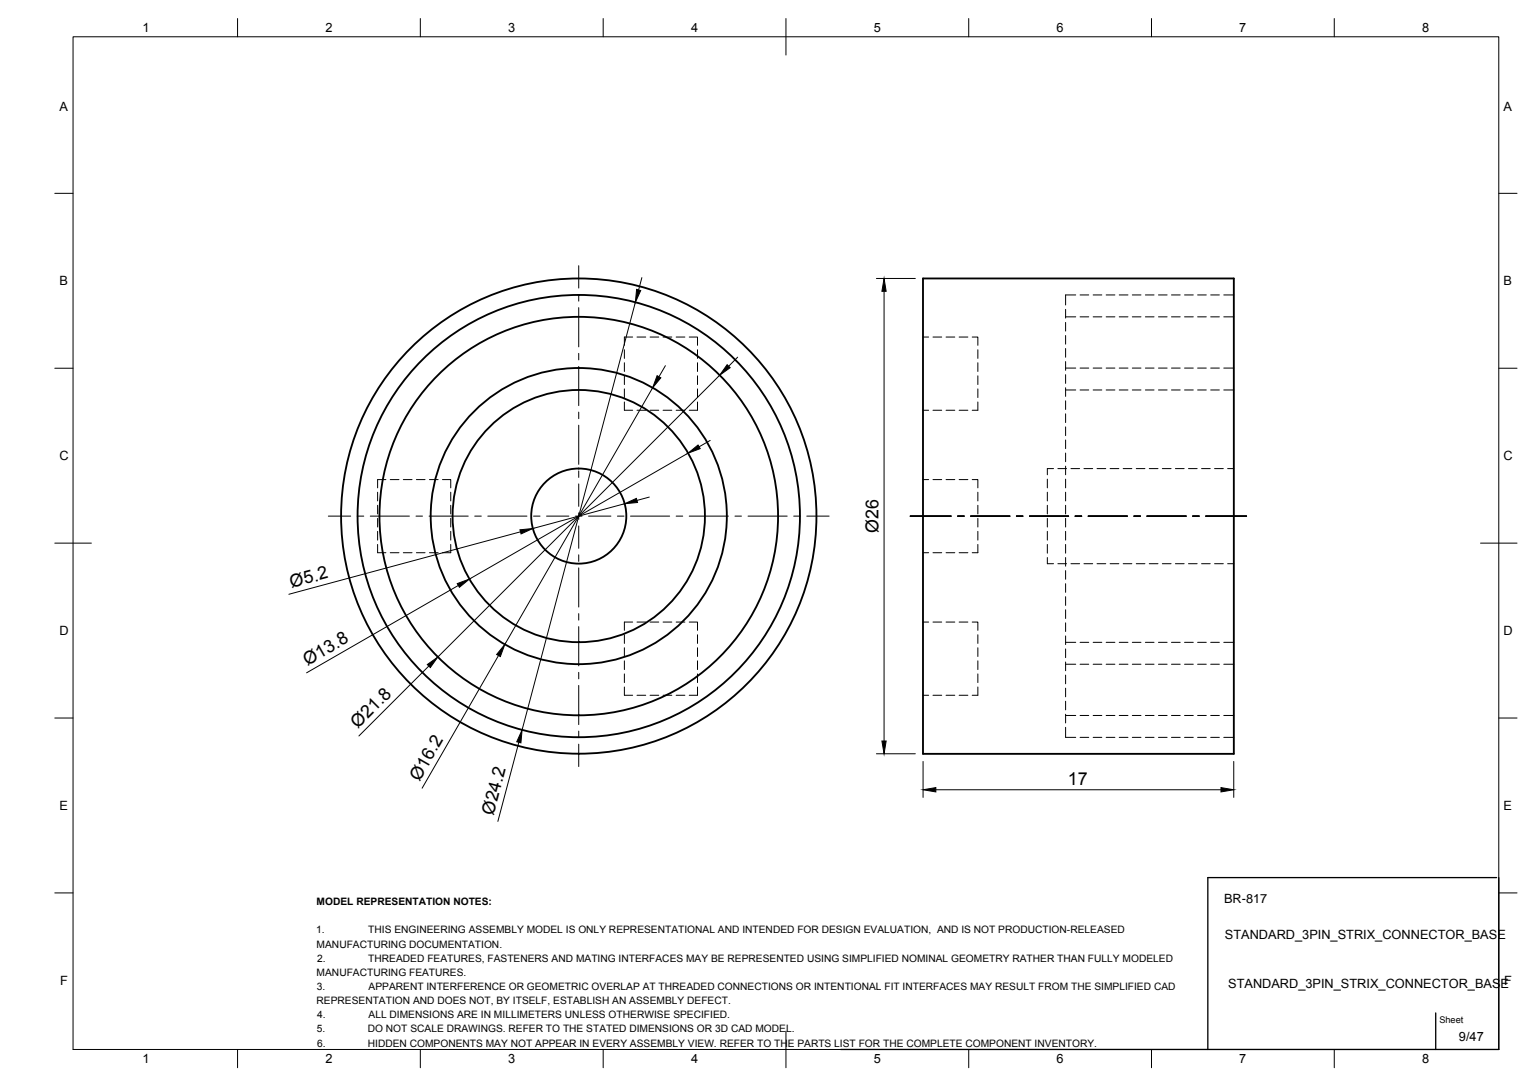
ISO-10303-21;
HEADER;
FILE_DESCRIPTION((''),'2;1');
FILE_NAME('STANDARD_3PIN_STRIX_CONNECTOR_BASE.step','2026-10-01T22:07:29-07:00',(''),(''),'','','');
FILE_SCHEMA (('AUTOMOTIVE_DESIGN { 1 0 10303 214 3 1 1 }'));
ENDSEC;
DATA;
#10=MECHANICAL_DESIGN_GEOMETRIC_PRESENTATION_REPRESENTATION('',(#545),#15484);
#475=SHAPE_REPRESENTATION_RELATIONSHIP('SRR','None',#15623,#510) ;
#510=ADVANCED_BREP_SHAPE_REPRESENTATION('',(#587),#15447) ;
#545=STYLED_ITEM('',(#15833),#587) ;
#587=MANIFOLD_SOLID_BREP('STANDARD_3PIN_STRIX_CONNECTOR_BASE',#8254) ;
#646=CYLINDRICAL_SURFACE('',#8800,0.26) ;
#647=CYLINDRICAL_SURFACE('',#8819,0.69) ;
#648=CYLINDRICAL_SURFACE('',#8822,0.81) ;
#649=CYLINDRICAL_SURFACE('',#8828,1.09) ;
#650=CYLINDRICAL_SURFACE('',#8830,1.21) ;
#651=CYLINDRICAL_SURFACE('',#8836,1.3) ;
#837=FACE_BOUND('',#1982,.T.) ;
#838=FACE_BOUND('',#1984,.T.) ;
#839=FACE_BOUND('',#1988,.T.) ;
#840=FACE_BOUND('',#1990,.T.) ;
#841=FACE_BOUND('',#1993,.T.) ;
#842=FACE_BOUND('',#1995,.T.) ;
#843=FACE_BOUND('',#1996,.T.) ;
#844=FACE_BOUND('',#1997,.T.) ;
#925=CIRCLE('',#8801,0.26) ;
#926=CIRCLE('',#8802,0.26) ;
#927=CIRCLE('',#8820,0.69) ;
#928=CIRCLE('',#8821,0.69) ;
#929=CIRCLE('',#8823,0.81) ;
#930=CIRCLE('',#8824,0.81) ;
#931=CIRCLE('',#8827,1.09) ;
#932=CIRCLE('',#8829,1.09) ;
#933=CIRCLE('',#8831,1.21) ;
#934=CIRCLE('',#8832,1.21) ;
#935=CIRCLE('',#8835,1.3) ;
#936=CIRCLE('',#8837,1.3) ;
#1435=FACE_OUTER_BOUND('',#1962,.T.) ;
#1436=FACE_OUTER_BOUND('',#1963,.T.) ;
#1437=FACE_OUTER_BOUND('',#1964,.T.) ;
#1438=FACE_OUTER_BOUND('',#1965,.T.) ;
#1439=FACE_OUTER_BOUND('',#1966,.T.) ;
#1440=FACE_OUTER_BOUND('',#1967,.T.) ;
#1441=FACE_OUTER_BOUND('',#1968,.T.) ;
#1442=FACE_OUTER_BOUND('',#1969,.T.) ;
#1443=FACE_OUTER_BOUND('',#1970,.T.) ;
#1444=FACE_OUTER_BOUND('',#1971,.T.) ;
#1445=FACE_OUTER_BOUND('',#1972,.T.) ;
#1446=FACE_OUTER_BOUND('',#1973,.T.) ;
#1447=FACE_OUTER_BOUND('',#1974,.T.) ;
#1448=FACE_OUTER_BOUND('',#1975,.T.) ;
#1449=FACE_OUTER_BOUND('',#1976,.T.) ;
#1450=FACE_OUTER_BOUND('',#1977,.T.) ;
#1451=FACE_OUTER_BOUND('',#1978,.T.) ;
#1452=FACE_OUTER_BOUND('',#1979,.T.) ;
#1453=FACE_OUTER_BOUND('',#1980,.T.) ;
#1454=FACE_OUTER_BOUND('',#1981,.T.) ;
#1455=FACE_OUTER_BOUND('',#1983,.T.) ;
#1456=FACE_OUTER_BOUND('',#1985,.T.) ;
#1457=FACE_OUTER_BOUND('',#1986,.T.) ;
#1458=FACE_OUTER_BOUND('',#1987,.T.) ;
#1459=FACE_OUTER_BOUND('',#1989,.T.) ;
#1460=FACE_OUTER_BOUND('',#1991,.T.) ;
#1461=FACE_OUTER_BOUND('',#1992,.T.) ;
#1462=FACE_OUTER_BOUND('',#1994,.T.) ;
#1962=EDGE_LOOP('',(#5603,#5604,#5605,#5606)) ;
#1963=EDGE_LOOP('',(#5607)) ;
#1964=EDGE_LOOP('',(#5608,#5609,#5610,#5611)) ;
#1965=EDGE_LOOP('',(#5612,#5613,#5614,#5615)) ;
#1966=EDGE_LOOP('',(#5616,#5617,#5618,#5619)) ;
#1967=EDGE_LOOP('',(#5620,#5621,#5622,#5623)) ;
#1968=EDGE_LOOP('',(#5624,#5625,#5626,#5627)) ;
#1969=EDGE_LOOP('',(#5628,#5629,#5630,#5631)) ;
#1970=EDGE_LOOP('',(#5632,#5633,#5634,#5635)) ;
#1971=EDGE_LOOP('',(#5636,#5637,#5638,#5639)) ;
#1972=EDGE_LOOP('',(#5640,#5641,#5642,#5643)) ;
#1973=EDGE_LOOP('',(#5644,#5645,#5646,#5647)) ;
#1974=EDGE_LOOP('',(#5648,#5649,#5650,#5651)) ;
#1975=EDGE_LOOP('',(#5652,#5653,#5654,#5655)) ;
#1976=EDGE_LOOP('',(#5656,#5657,#5658,#5659)) ;
#1977=EDGE_LOOP('',(#5660,#5661,#5662,#5663)) ;
#1978=EDGE_LOOP('',(#5664,#5665,#5666,#5667)) ;
#1979=EDGE_LOOP('',(#5668,#5669,#5670,#5671)) ;
#1980=EDGE_LOOP('',(#5672,#5673,#5674,#5675)) ;
#1981=EDGE_LOOP('',(#5676)) ;
#1982=EDGE_LOOP('',(#5677)) ;
#1983=EDGE_LOOP('',(#5678)) ;
#1984=EDGE_LOOP('',(#5679)) ;
#1985=EDGE_LOOP('',(#5680,#5681,#5682,#5683)) ;
#1986=EDGE_LOOP('',(#5684,#5685,#5686,#5687)) ;
#1987=EDGE_LOOP('',(#5688)) ;
#1988=EDGE_LOOP('',(#5689)) ;
#1989=EDGE_LOOP('',(#5690)) ;
#1990=EDGE_LOOP('',(#5691)) ;
#1991=EDGE_LOOP('',(#5692,#5693,#5694,#5695)) ;
#1992=EDGE_LOOP('',(#5696)) ;
#1993=EDGE_LOOP('',(#5697)) ;
#1994=EDGE_LOOP('',(#5698)) ;
#1995=EDGE_LOOP('',(#5699,#5700,#5701,#5702)) ;
#1996=EDGE_LOOP('',(#5703,#5704,#5705,#5706)) ;
#1997=EDGE_LOOP('',(#5707,#5708,#5709,#5710)) ;
#2565=LINE('',#13242,#3039) ;
#2566=LINE('',#13248,#3040) ;
#2567=LINE('',#13250,#3041) ;
#2568=LINE('',#13252,#3042) ;
#2569=LINE('',#13253,#3043) ;
#2570=LINE('',#13256,#3044) ;
#2571=LINE('',#13258,#3045) ;
#2572=LINE('',#13259,#3046) ;
#2573=LINE('',#13262,#3047) ;
#2574=LINE('',#13263,#3048) ;
#2575=LINE('',#13266,#3049) ;
#2576=LINE('',#13267,#3050) ;
#2577=LINE('',#13269,#3051) ;
#2578=LINE('',#13273,#3052) ;
#2579=LINE('',#13275,#3053) ;
#2580=LINE('',#13277,#3054) ;
#2581=LINE('',#13278,#3055) ;
#2582=LINE('',#13281,#3056) ;
#2583=LINE('',#13283,#3057) ;
#2584=LINE('',#13284,#3058) ;
#2585=LINE('',#13287,#3059) ;
#2586=LINE('',#13288,#3060) ;
#2587=LINE('',#13291,#3061) ;
#2588=LINE('',#13292,#3062) ;
#2589=LINE('',#13294,#3063) ;
#2590=LINE('',#13298,#3064) ;
#2591=LINE('',#13300,#3065) ;
#2592=LINE('',#13302,#3066) ;
#2593=LINE('',#13303,#3067) ;
#2594=LINE('',#13306,#3068) ;
#2595=LINE('',#13308,#3069) ;
#2596=LINE('',#13309,#3070) ;
#2597=LINE('',#13312,#3071) ;
#2598=LINE('',#13313,#3072) ;
#2599=LINE('',#13316,#3073) ;
#2600=LINE('',#13317,#3074) ;
#2601=LINE('',#13319,#3075) ;
#2602=LINE('',#13324,#3076) ;
#2603=LINE('',#13330,#3077) ;
#2604=LINE('',#13339,#3078) ;
#2605=LINE('',#13344,#3079) ;
#2606=LINE('',#13353,#3080) ;
#3039=VECTOR('',#10290,0.26) ;
#3040=VECTOR('',#10297,1.) ;
#3041=VECTOR('',#10298,1.) ;
#3042=VECTOR('',#10299,1.) ;
#3043=VECTOR('',#10300,1.) ;
#3044=VECTOR('',#10303,1.) ;
#3045=VECTOR('',#10304,1.) ;
#3046=VECTOR('',#10305,1.) ;
#3047=VECTOR('',#10308,1.) ;
#3048=VECTOR('',#10309,1.) ;
#3049=VECTOR('',#10312,1.) ;
#3050=VECTOR('',#10313,1.) ;
#3051=VECTOR('',#10316,1.) ;
#3052=VECTOR('',#10319,1.) ;
#3053=VECTOR('',#10320,1.) ;
#3054=VECTOR('',#10321,1.) ;
#3055=VECTOR('',#10322,1.) ;
#3056=VECTOR('',#10325,1.) ;
#3057=VECTOR('',#10326,1.) ;
#3058=VECTOR('',#10327,1.) ;
#3059=VECTOR('',#10330,1.) ;
#3060=VECTOR('',#10331,1.) ;
#3061=VECTOR('',#10334,1.) ;
#3062=VECTOR('',#10335,1.) ;
#3063=VECTOR('',#10338,1.) ;
#3064=VECTOR('',#10341,1.) ;
#3065=VECTOR('',#10342,1.) ;
#3066=VECTOR('',#10343,1.) ;
#3067=VECTOR('',#10344,1.) ;
#3068=VECTOR('',#10347,1.) ;
#3069=VECTOR('',#10348,1.) ;
#3070=VECTOR('',#10349,1.) ;
#3071=VECTOR('',#10352,1.) ;
#3072=VECTOR('',#10353,1.) ;
#3073=VECTOR('',#10356,1.) ;
#3074=VECTOR('',#10357,1.) ;
#3075=VECTOR('',#10360,1.) ;
#3076=VECTOR('',#10365,0.69) ;
#3077=VECTOR('',#10372,0.81) ;
#3078=VECTOR('',#10385,1.09) ;
#3079=VECTOR('',#10390,1.21) ;
#3080=VECTOR('',#10403,1.3) ;
#3498=VERTEX_POINT('',#13239) ;
#3499=VERTEX_POINT('',#13241) ;
#3500=VERTEX_POINT('',#13246) ;
#3501=VERTEX_POINT('',#13247) ;
#3502=VERTEX_POINT('',#13249) ;
#3503=VERTEX_POINT('',#13251) ;
#3504=VERTEX_POINT('',#13255) ;
#3505=VERTEX_POINT('',#13257) ;
#3506=VERTEX_POINT('',#13261) ;
#3507=VERTEX_POINT('',#13265) ;
#3508=VERTEX_POINT('',#13271) ;
#3509=VERTEX_POINT('',#13272) ;
#3510=VERTEX_POINT('',#13274) ;
#3511=VERTEX_POINT('',#13276) ;
#3512=VERTEX_POINT('',#13280) ;
#3513=VERTEX_POINT('',#13282) ;
#3514=VERTEX_POINT('',#13286) ;
#3515=VERTEX_POINT('',#13290) ;
#3516=VERTEX_POINT('',#13296) ;
#3517=VERTEX_POINT('',#13297) ;
#3518=VERTEX_POINT('',#13299) ;
#3519=VERTEX_POINT('',#13301) ;
#3520=VERTEX_POINT('',#13305) ;
#3521=VERTEX_POINT('',#13307) ;
#3522=VERTEX_POINT('',#13311) ;
#3523=VERTEX_POINT('',#13315) ;
#3524=VERTEX_POINT('',#13321) ;
#3525=VERTEX_POINT('',#13323) ;
#3526=VERTEX_POINT('',#13327) ;
#3527=VERTEX_POINT('',#13329) ;
#3528=VERTEX_POINT('',#13334) ;
#3529=VERTEX_POINT('',#13337) ;
#3530=VERTEX_POINT('',#13341) ;
#3531=VERTEX_POINT('',#13343) ;
#3532=VERTEX_POINT('',#13348) ;
#3533=VERTEX_POINT('',#13351) ;
#4306=EDGE_CURVE('',#3498,#3498,#925,.T.) ;
#4307=EDGE_CURVE('',#3498,#3499,#2565,.T.) ;
#4308=EDGE_CURVE('',#3499,#3499,#926,.T.) ;
#4309=EDGE_CURVE('',#3500,#3501,#2566,.T.) ;
#4310=EDGE_CURVE('',#3500,#3502,#2567,.T.) ;
#4311=EDGE_CURVE('',#3502,#3503,#2568,.T.) ;
#4312=EDGE_CURVE('',#3501,#3503,#2569,.T.) ;
#4313=EDGE_CURVE('',#3501,#3504,#2570,.T.) ;
#4314=EDGE_CURVE('',#3503,#3505,#2571,.T.) ;
#4315=EDGE_CURVE('',#3504,#3505,#2572,.T.) ;
#4316=EDGE_CURVE('',#3506,#3502,#2573,.T.) ;
#4317=EDGE_CURVE('',#3505,#3506,#2574,.T.) ;
#4318=EDGE_CURVE('',#3504,#3507,#2575,.T.) ;
#4319=EDGE_CURVE('',#3507,#3506,#2576,.T.) ;
#4320=EDGE_CURVE('',#3507,#3500,#2577,.T.) ;
#4321=EDGE_CURVE('',#3508,#3509,#2578,.T.) ;
#4322=EDGE_CURVE('',#3508,#3510,#2579,.T.) ;
#4323=EDGE_CURVE('',#3510,#3511,#2580,.T.) ;
#4324=EDGE_CURVE('',#3509,#3511,#2581,.T.) ;
#4325=EDGE_CURVE('',#3509,#3512,#2582,.T.) ;
#4326=EDGE_CURVE('',#3511,#3513,#2583,.T.) ;
#4327=EDGE_CURVE('',#3512,#3513,#2584,.T.) ;
#4328=EDGE_CURVE('',#3514,#3510,#2585,.T.) ;
#4329=EDGE_CURVE('',#3513,#3514,#2586,.T.) ;
#4330=EDGE_CURVE('',#3512,#3515,#2587,.T.) ;
#4331=EDGE_CURVE('',#3515,#3514,#2588,.T.) ;
#4332=EDGE_CURVE('',#3515,#3508,#2589,.T.) ;
#4333=EDGE_CURVE('',#3516,#3517,#2590,.T.) ;
#4334=EDGE_CURVE('',#3516,#3518,#2591,.T.) ;
#4335=EDGE_CURVE('',#3518,#3519,#2592,.T.) ;
#4336=EDGE_CURVE('',#3517,#3519,#2593,.T.) ;
#4337=EDGE_CURVE('',#3517,#3520,#2594,.T.) ;
#4338=EDGE_CURVE('',#3519,#3521,#2595,.T.) ;
#4339=EDGE_CURVE('',#3520,#3521,#2596,.T.) ;
#4340=EDGE_CURVE('',#3522,#3518,#2597,.T.) ;
#4341=EDGE_CURVE('',#3521,#3522,#2598,.T.) ;
#4342=EDGE_CURVE('',#3520,#3523,#2599,.T.) ;
#4343=EDGE_CURVE('',#3523,#3522,#2600,.T.) ;
#4344=EDGE_CURVE('',#3523,#3516,#2601,.T.) ;
#4345=EDGE_CURVE('',#3524,#3524,#927,.T.) ;
#4346=EDGE_CURVE('',#3524,#3525,#2602,.T.) ;
#4347=EDGE_CURVE('',#3525,#3525,#928,.T.) ;
#4348=EDGE_CURVE('',#3526,#3526,#929,.T.) ;
#4349=EDGE_CURVE('',#3526,#3527,#2603,.T.) ;
#4350=EDGE_CURVE('',#3527,#3527,#930,.T.) ;
#4351=EDGE_CURVE('',#3528,#3528,#931,.T.) ;
#4352=EDGE_CURVE('',#3529,#3529,#932,.T.) ;
#4353=EDGE_CURVE('',#3529,#3528,#2604,.T.) ;
#4354=EDGE_CURVE('',#3530,#3530,#933,.T.) ;
#4355=EDGE_CURVE('',#3530,#3531,#2605,.T.) ;
#4356=EDGE_CURVE('',#3531,#3531,#934,.T.) ;
#4357=EDGE_CURVE('',#3532,#3532,#935,.T.) ;
#4358=EDGE_CURVE('',#3533,#3533,#936,.T.) ;
#4359=EDGE_CURVE('',#3533,#3532,#2606,.T.) ;
#5603=ORIENTED_EDGE('',*,*,#4306,.F.) ;
#5604=ORIENTED_EDGE('',*,*,#4307,.T.) ;
#5605=ORIENTED_EDGE('',*,*,#4308,.T.) ;
#5606=ORIENTED_EDGE('',*,*,#4307,.F.) ;
#5607=ORIENTED_EDGE('',*,*,#4308,.F.) ;
#5608=ORIENTED_EDGE('',*,*,#4309,.F.) ;
#5609=ORIENTED_EDGE('',*,*,#4310,.T.) ;
#5610=ORIENTED_EDGE('',*,*,#4311,.T.) ;
#5611=ORIENTED_EDGE('',*,*,#4312,.F.) ;
#5612=ORIENTED_EDGE('',*,*,#4313,.F.) ;
#5613=ORIENTED_EDGE('',*,*,#4312,.T.) ;
#5614=ORIENTED_EDGE('',*,*,#4314,.T.) ;
#5615=ORIENTED_EDGE('',*,*,#4315,.F.) ;
#5616=ORIENTED_EDGE('',*,*,#4314,.F.) ;
#5617=ORIENTED_EDGE('',*,*,#4311,.F.) ;
#5618=ORIENTED_EDGE('',*,*,#4316,.F.) ;
#5619=ORIENTED_EDGE('',*,*,#4317,.F.) ;
#5620=ORIENTED_EDGE('',*,*,#4318,.F.) ;
#5621=ORIENTED_EDGE('',*,*,#4315,.T.) ;
#5622=ORIENTED_EDGE('',*,*,#4317,.T.) ;
#5623=ORIENTED_EDGE('',*,*,#4319,.F.) ;
#5624=ORIENTED_EDGE('',*,*,#4320,.F.) ;
#5625=ORIENTED_EDGE('',*,*,#4319,.T.) ;
#5626=ORIENTED_EDGE('',*,*,#4316,.T.) ;
#5627=ORIENTED_EDGE('',*,*,#4310,.F.) ;
#5628=ORIENTED_EDGE('',*,*,#4321,.F.) ;
#5629=ORIENTED_EDGE('',*,*,#4322,.T.) ;
#5630=ORIENTED_EDGE('',*,*,#4323,.T.) ;
#5631=ORIENTED_EDGE('',*,*,#4324,.F.) ;
#5632=ORIENTED_EDGE('',*,*,#4325,.F.) ;
#5633=ORIENTED_EDGE('',*,*,#4324,.T.) ;
#5634=ORIENTED_EDGE('',*,*,#4326,.T.) ;
#5635=ORIENTED_EDGE('',*,*,#4327,.F.) ;
#5636=ORIENTED_EDGE('',*,*,#4326,.F.) ;
#5637=ORIENTED_EDGE('',*,*,#4323,.F.) ;
#5638=ORIENTED_EDGE('',*,*,#4328,.F.) ;
#5639=ORIENTED_EDGE('',*,*,#4329,.F.) ;
#5640=ORIENTED_EDGE('',*,*,#4330,.F.) ;
#5641=ORIENTED_EDGE('',*,*,#4327,.T.) ;
#5642=ORIENTED_EDGE('',*,*,#4329,.T.) ;
#5643=ORIENTED_EDGE('',*,*,#4331,.F.) ;
#5644=ORIENTED_EDGE('',*,*,#4332,.F.) ;
#5645=ORIENTED_EDGE('',*,*,#4331,.T.) ;
#5646=ORIENTED_EDGE('',*,*,#4328,.T.) ;
#5647=ORIENTED_EDGE('',*,*,#4322,.F.) ;
#5648=ORIENTED_EDGE('',*,*,#4333,.F.) ;
#5649=ORIENTED_EDGE('',*,*,#4334,.T.) ;
#5650=ORIENTED_EDGE('',*,*,#4335,.T.) ;
#5651=ORIENTED_EDGE('',*,*,#4336,.F.) ;
#5652=ORIENTED_EDGE('',*,*,#4337,.F.) ;
#5653=ORIENTED_EDGE('',*,*,#4336,.T.) ;
#5654=ORIENTED_EDGE('',*,*,#4338,.T.) ;
#5655=ORIENTED_EDGE('',*,*,#4339,.F.) ;
#5656=ORIENTED_EDGE('',*,*,#4338,.F.) ;
#5657=ORIENTED_EDGE('',*,*,#4335,.F.) ;
#5658=ORIENTED_EDGE('',*,*,#4340,.F.) ;
#5659=ORIENTED_EDGE('',*,*,#4341,.F.) ;
#5660=ORIENTED_EDGE('',*,*,#4342,.F.) ;
#5661=ORIENTED_EDGE('',*,*,#4339,.T.) ;
#5662=ORIENTED_EDGE('',*,*,#4341,.T.) ;
#5663=ORIENTED_EDGE('',*,*,#4343,.F.) ;
#5664=ORIENTED_EDGE('',*,*,#4344,.F.) ;
#5665=ORIENTED_EDGE('',*,*,#4343,.T.) ;
#5666=ORIENTED_EDGE('',*,*,#4340,.T.) ;
#5667=ORIENTED_EDGE('',*,*,#4334,.F.) ;
#5668=ORIENTED_EDGE('',*,*,#4345,.T.) ;
#5669=ORIENTED_EDGE('',*,*,#4346,.T.) ;
#5670=ORIENTED_EDGE('',*,*,#4347,.F.) ;
#5671=ORIENTED_EDGE('',*,*,#4346,.F.) ;
#5672=ORIENTED_EDGE('',*,*,#4348,.F.) ;
#5673=ORIENTED_EDGE('',*,*,#4349,.T.) ;
#5674=ORIENTED_EDGE('',*,*,#4350,.T.) ;
#5675=ORIENTED_EDGE('',*,*,#4349,.F.) ;
#5676=ORIENTED_EDGE('',*,*,#4350,.F.) ;
#5677=ORIENTED_EDGE('',*,*,#4345,.F.) ;
#5678=ORIENTED_EDGE('',*,*,#4351,.T.) ;
#5679=ORIENTED_EDGE('',*,*,#4348,.T.) ;
#5680=ORIENTED_EDGE('',*,*,#4352,.T.) ;
#5681=ORIENTED_EDGE('',*,*,#4353,.T.) ;
#5682=ORIENTED_EDGE('',*,*,#4351,.F.) ;
#5683=ORIENTED_EDGE('',*,*,#4353,.F.) ;
#5684=ORIENTED_EDGE('',*,*,#4354,.F.) ;
#5685=ORIENTED_EDGE('',*,*,#4355,.T.) ;
#5686=ORIENTED_EDGE('',*,*,#4356,.T.) ;
#5687=ORIENTED_EDGE('',*,*,#4355,.F.) ;
#5688=ORIENTED_EDGE('',*,*,#4356,.F.) ;
#5689=ORIENTED_EDGE('',*,*,#4352,.F.) ;
#5690=ORIENTED_EDGE('',*,*,#4357,.T.) ;
#5691=ORIENTED_EDGE('',*,*,#4354,.T.) ;
#5692=ORIENTED_EDGE('',*,*,#4358,.F.) ;
#5693=ORIENTED_EDGE('',*,*,#4359,.T.) ;
#5694=ORIENTED_EDGE('',*,*,#4357,.F.) ;
#5695=ORIENTED_EDGE('',*,*,#4359,.F.) ;
#5696=ORIENTED_EDGE('',*,*,#4347,.T.) ;
#5697=ORIENTED_EDGE('',*,*,#4306,.T.) ;
#5698=ORIENTED_EDGE('',*,*,#4358,.T.) ;
#5699=ORIENTED_EDGE('',*,*,#4318,.T.) ;
#5700=ORIENTED_EDGE('',*,*,#4320,.T.) ;
#5701=ORIENTED_EDGE('',*,*,#4309,.T.) ;
#5702=ORIENTED_EDGE('',*,*,#4313,.T.) ;
#5703=ORIENTED_EDGE('',*,*,#4330,.T.) ;
#5704=ORIENTED_EDGE('',*,*,#4332,.T.) ;
#5705=ORIENTED_EDGE('',*,*,#4321,.T.) ;
#5706=ORIENTED_EDGE('',*,*,#4325,.T.) ;
#5707=ORIENTED_EDGE('',*,*,#4342,.T.) ;
#5708=ORIENTED_EDGE('',*,*,#4344,.T.) ;
#5709=ORIENTED_EDGE('',*,*,#4333,.T.) ;
#5710=ORIENTED_EDGE('',*,*,#4337,.T.) ;
#7587=PLANE('',#8803) ;
#7588=PLANE('',#8804) ;
#7589=PLANE('',#8805) ;
#7590=PLANE('',#8806) ;
#7591=PLANE('',#8807) ;
#7592=PLANE('',#8808) ;
#7593=PLANE('',#8809) ;
#7594=PLANE('',#8810) ;
#7595=PLANE('',#8811) ;
#7596=PLANE('',#8812) ;
#7597=PLANE('',#8813) ;
#7598=PLANE('',#8814) ;
#7599=PLANE('',#8815) ;
#7600=PLANE('',#8816) ;
#7601=PLANE('',#8817) ;
#7602=PLANE('',#8818) ;
#7603=PLANE('',#8825) ;
#7604=PLANE('',#8826) ;
#7605=PLANE('',#8833) ;
#7606=PLANE('',#8834) ;
#7607=PLANE('',#8838) ;
#7608=PLANE('',#8839) ;
#7822=ADVANCED_FACE('',(#1435),#646,.F.) ;
#7823=ADVANCED_FACE('',(#1436),#7587,.F.) ;
#7824=ADVANCED_FACE('',(#1437),#7588,.T.) ;
#7825=ADVANCED_FACE('',(#1438),#7589,.T.) ;
#7826=ADVANCED_FACE('',(#1439),#7590,.T.) ;
#7827=ADVANCED_FACE('',(#1440),#7591,.T.) ;
#7828=ADVANCED_FACE('',(#1441),#7592,.T.) ;
#7829=ADVANCED_FACE('',(#1442),#7593,.T.) ;
#7830=ADVANCED_FACE('',(#1443),#7594,.T.) ;
#7831=ADVANCED_FACE('',(#1444),#7595,.T.) ;
#7832=ADVANCED_FACE('',(#1445),#7596,.T.) ;
#7833=ADVANCED_FACE('',(#1446),#7597,.T.) ;
#7834=ADVANCED_FACE('',(#1447),#7598,.T.) ;
#7835=ADVANCED_FACE('',(#1448),#7599,.T.) ;
#7836=ADVANCED_FACE('',(#1449),#7600,.T.) ;
#7837=ADVANCED_FACE('',(#1450),#7601,.T.) ;
#7838=ADVANCED_FACE('',(#1451),#7602,.T.) ;
#7839=ADVANCED_FACE('',(#1452),#647,.T.) ;
#7840=ADVANCED_FACE('',(#1453),#648,.F.) ;
#7841=ADVANCED_FACE('',(#1454,#837),#7603,.F.) ;
#7842=ADVANCED_FACE('',(#1455,#838),#7604,.T.) ;
#7843=ADVANCED_FACE('',(#1456),#649,.T.) ;
#7844=ADVANCED_FACE('',(#1457),#650,.F.) ;
#7845=ADVANCED_FACE('',(#1458,#839),#7605,.F.) ;
#7846=ADVANCED_FACE('',(#1459,#840),#7606,.T.) ;
#7847=ADVANCED_FACE('',(#1460),#651,.T.) ;
#7848=ADVANCED_FACE('',(#1461,#841),#7607,.T.) ;
#7849=ADVANCED_FACE('',(#1462,#842,#843,#844),#7608,.T.) ;
#8254=CLOSED_SHELL('',(#7822,#7823,#7824,#7825,#7826,#7827,#7828,#7829,
#7830,#7831,#7832,#7833,#7834,#7835,#7836,#7837,#7838,#7839,#7840,#7841,
#7842,#7843,#7844,#7845,#7846,#7847,#7848,#7849)) ;
#8799=AXIS2_PLACEMENT_3D('',#13237,#10284,#10285) ;
#8800=AXIS2_PLACEMENT_3D('',#13238,#10286,#10287) ;
#8801=AXIS2_PLACEMENT_3D('',#13240,#10288,#10289) ;
#8802=AXIS2_PLACEMENT_3D('',#13243,#10291,#10292) ;
#8803=AXIS2_PLACEMENT_3D('',#13244,#10293,#10294) ;
#8804=AXIS2_PLACEMENT_3D('',#13245,#10295,#10296) ;
#8805=AXIS2_PLACEMENT_3D('',#13254,#10301,#10302) ;
#8806=AXIS2_PLACEMENT_3D('',#13260,#10306,#10307) ;
#8807=AXIS2_PLACEMENT_3D('',#13264,#10310,#10311) ;
#8808=AXIS2_PLACEMENT_3D('',#13268,#10314,#10315) ;
#8809=AXIS2_PLACEMENT_3D('',#13270,#10317,#10318) ;
#8810=AXIS2_PLACEMENT_3D('',#13279,#10323,#10324) ;
#8811=AXIS2_PLACEMENT_3D('',#13285,#10328,#10329) ;
#8812=AXIS2_PLACEMENT_3D('',#13289,#10332,#10333) ;
#8813=AXIS2_PLACEMENT_3D('',#13293,#10336,#10337) ;
#8814=AXIS2_PLACEMENT_3D('',#13295,#10339,#10340) ;
#8815=AXIS2_PLACEMENT_3D('',#13304,#10345,#10346) ;
#8816=AXIS2_PLACEMENT_3D('',#13310,#10350,#10351) ;
#8817=AXIS2_PLACEMENT_3D('',#13314,#10354,#10355) ;
#8818=AXIS2_PLACEMENT_3D('',#13318,#10358,#10359) ;
#8819=AXIS2_PLACEMENT_3D('',#13320,#10361,#10362) ;
#8820=AXIS2_PLACEMENT_3D('',#13322,#10363,#10364) ;
#8821=AXIS2_PLACEMENT_3D('',#13325,#10366,#10367) ;
#8822=AXIS2_PLACEMENT_3D('',#13326,#10368,#10369) ;
#8823=AXIS2_PLACEMENT_3D('',#13328,#10370,#10371) ;
#8824=AXIS2_PLACEMENT_3D('',#13331,#10373,#10374) ;
#8825=AXIS2_PLACEMENT_3D('',#13332,#10375,#10376) ;
#8826=AXIS2_PLACEMENT_3D('',#13333,#10377,#10378) ;
#8827=AXIS2_PLACEMENT_3D('',#13335,#10379,#10380) ;
#8828=AXIS2_PLACEMENT_3D('',#13336,#10381,#10382) ;
#8829=AXIS2_PLACEMENT_3D('',#13338,#10383,#10384) ;
#8830=AXIS2_PLACEMENT_3D('',#13340,#10386,#10387) ;
#8831=AXIS2_PLACEMENT_3D('',#13342,#10388,#10389) ;
#8832=AXIS2_PLACEMENT_3D('',#13345,#10391,#10392) ;
#8833=AXIS2_PLACEMENT_3D('',#13346,#10393,#10394) ;
#8834=AXIS2_PLACEMENT_3D('',#13347,#10395,#10396) ;
#8835=AXIS2_PLACEMENT_3D('',#13349,#10397,#10398) ;
#8836=AXIS2_PLACEMENT_3D('',#13350,#10399,#10400) ;
#8837=AXIS2_PLACEMENT_3D('',#13352,#10401,#10402) ;
#8838=AXIS2_PLACEMENT_3D('',#13354,#10404,#10405) ;
#8839=AXIS2_PLACEMENT_3D('',#13355,#10406,#10407) ;
#10284=DIRECTION('axis',(0.,0.,1.)) ;
#10285=DIRECTION('refdir',(1.,0.,0.)) ;
#10286=DIRECTION('center_axis',(0.,0.,1.)) ;
#10287=DIRECTION('ref_axis',(1.,0.,0.)) ;
#10288=DIRECTION('center_axis',(0.,0.,1.)) ;
#10289=DIRECTION('ref_axis',(1.,0.,0.)) ;
#10290=DIRECTION('',(0.,0.,1.)) ;
#10291=DIRECTION('center_axis',(0.,0.,1.)) ;
#10292=DIRECTION('ref_axis',(1.,0.,0.)) ;
#10293=DIRECTION('center_axis',(0.,0.,1.)) ;
#10294=DIRECTION('ref_axis',(1.,0.,0.)) ;
#10295=DIRECTION('center_axis',(0.,-1.,0.)) ;
#10296=DIRECTION('ref_axis',(0.,0.,-1.)) ;
#10297=DIRECTION('',(1.,0.,0.)) ;
#10298=DIRECTION('',(0.,0.,-1.)) ;
#10299=DIRECTION('',(1.,0.,0.)) ;
#10300=DIRECTION('',(0.,0.,-1.)) ;
#10301=DIRECTION('center_axis',(-1.,0.,0.)) ;
#10302=DIRECTION('ref_axis',(0.,0.,1.)) ;
#10303=DIRECTION('',(0.,-1.,0.)) ;
#10304=DIRECTION('',(0.,-1.,0.)) ;
#10305=DIRECTION('',(0.,0.,-1.)) ;
#10306=DIRECTION('center_axis',(0.,0.,1.)) ;
#10307=DIRECTION('ref_axis',(1.,0.,0.)) ;
#10308=DIRECTION('',(0.,1.,0.)) ;
#10309=DIRECTION('',(-1.,0.,0.)) ;
#10310=DIRECTION('center_axis',(0.,1.,0.)) ;
#10311=DIRECTION('ref_axis',(0.,0.,1.)) ;
#10312=DIRECTION('',(-1.,0.,0.)) ;
#10313=DIRECTION('',(0.,0.,-1.)) ;
#10314=DIRECTION('center_axis',(1.,0.,0.)) ;
#10315=DIRECTION('ref_axis',(0.,0.,-1.)) ;
#10316=DIRECTION('',(0.,1.,0.)) ;
#10317=DIRECTION('center_axis',(0.,-1.,0.)) ;
#10318=DIRECTION('ref_axis',(0.,0.,-1.)) ;
#10319=DIRECTION('',(1.,0.,0.)) ;
#10320=DIRECTION('',(0.,0.,-1.)) ;
#10321=DIRECTION('',(1.,0.,0.)) ;
#10322=DIRECTION('',(0.,0.,-1.)) ;
#10323=DIRECTION('center_axis',(-1.,0.,0.)) ;
#10324=DIRECTION('ref_axis',(0.,0.,1.)) ;
#10325=DIRECTION('',(0.,-1.,0.)) ;
#10326=DIRECTION('',(0.,-1.,0.)) ;
#10327=DIRECTION('',(0.,0.,-1.)) ;
#10328=DIRECTION('center_axis',(0.,0.,1.)) ;
#10329=DIRECTION('ref_axis',(1.,0.,0.)) ;
#10330=DIRECTION('',(0.,1.,0.)) ;
#10331=DIRECTION('',(-1.,0.,0.)) ;
#10332=DIRECTION('center_axis',(0.,1.,0.)) ;
#10333=DIRECTION('ref_axis',(0.,0.,1.)) ;
#10334=DIRECTION('',(-1.,0.,0.)) ;
#10335=DIRECTION('',(0.,0.,-1.)) ;
#10336=DIRECTION('center_axis',(1.,0.,0.)) ;
#10337=DIRECTION('ref_axis',(0.,0.,-1.)) ;
#10338=DIRECTION('',(0.,1.,0.)) ;
#10339=DIRECTION('center_axis',(0.,-1.,0.)) ;
#10340=DIRECTION('ref_axis',(0.,0.,-1.)) ;
#10341=DIRECTION('',(1.,0.,0.)) ;
#10342=DIRECTION('',(0.,0.,-1.)) ;
#10343=DIRECTION('',(1.,0.,0.)) ;
#10344=DIRECTION('',(0.,0.,-1.)) ;
#10345=DIRECTION('center_axis',(-1.,0.,0.)) ;
#10346=DIRECTION('ref_axis',(0.,0.,1.)) ;
#10347=DIRECTION('',(0.,-1.,0.)) ;
#10348=DIRECTION('',(0.,-1.,0.)) ;
#10349=DIRECTION('',(0.,0.,-1.)) ;
#10350=DIRECTION('center_axis',(0.,0.,1.)) ;
#10351=DIRECTION('ref_axis',(1.,0.,0.)) ;
#10352=DIRECTION('',(0.,1.,0.)) ;
#10353=DIRECTION('',(-1.,0.,0.)) ;
#10354=DIRECTION('center_axis',(0.,1.,0.)) ;
#10355=DIRECTION('ref_axis',(0.,0.,1.)) ;
#10356=DIRECTION('',(-1.,0.,0.)) ;
#10357=DIRECTION('',(0.,0.,-1.)) ;
#10358=DIRECTION('center_axis',(1.,0.,0.)) ;
#10359=DIRECTION('ref_axis',(0.,0.,-1.)) ;
#10360=DIRECTION('',(0.,1.,0.)) ;
#10361=DIRECTION('center_axis',(0.,0.,1.)) ;
#10362=DIRECTION('ref_axis',(1.,0.,0.)) ;
#10363=DIRECTION('center_axis',(0.,0.,-1.)) ;
#10364=DIRECTION('ref_axis',(1.,0.,0.)) ;
#10365=DIRECTION('',(0.,0.,-1.)) ;
#10366=DIRECTION('center_axis',(0.,0.,-1.)) ;
#10367=DIRECTION('ref_axis',(1.,0.,0.)) ;
#10368=DIRECTION('center_axis',(0.,0.,1.)) ;
#10369=DIRECTION('ref_axis',(1.,0.,0.)) ;
#10370=DIRECTION('center_axis',(0.,0.,1.)) ;
#10371=DIRECTION('ref_axis',(1.,0.,0.)) ;
#10372=DIRECTION('',(0.,0.,1.)) ;
#10373=DIRECTION('center_axis',(0.,0.,1.)) ;
#10374=DIRECTION('ref_axis',(1.,0.,0.)) ;
#10375=DIRECTION('center_axis',(0.,0.,1.)) ;
#10376=DIRECTION('ref_axis',(1.,0.,0.)) ;
#10377=DIRECTION('center_axis',(0.,0.,-1.)) ;
#10378=DIRECTION('ref_axis',(-1.,0.,0.)) ;
#10379=DIRECTION('center_axis',(0.,0.,-1.)) ;
#10380=DIRECTION('ref_axis',(1.,0.,0.)) ;
#10381=DIRECTION('center_axis',(0.,0.,1.)) ;
#10382=DIRECTION('ref_axis',(1.,0.,0.)) ;
#10383=DIRECTION('center_axis',(0.,0.,-1.)) ;
#10384=DIRECTION('ref_axis',(1.,0.,0.)) ;
#10385=DIRECTION('',(0.,0.,-1.)) ;
#10386=DIRECTION('center_axis',(0.,0.,1.)) ;
#10387=DIRECTION('ref_axis',(1.,0.,0.)) ;
#10388=DIRECTION('center_axis',(0.,0.,1.)) ;
#10389=DIRECTION('ref_axis',(1.,0.,0.)) ;
#10390=DIRECTION('',(0.,0.,1.)) ;
#10391=DIRECTION('center_axis',(0.,0.,1.)) ;
#10392=DIRECTION('ref_axis',(1.,0.,0.)) ;
#10393=DIRECTION('center_axis',(0.,0.,1.)) ;
#10394=DIRECTION('ref_axis',(1.,0.,0.)) ;
#10395=DIRECTION('center_axis',(0.,0.,-1.)) ;
#10396=DIRECTION('ref_axis',(-1.,0.,0.)) ;
#10397=DIRECTION('center_axis',(0.,0.,-1.)) ;
#10398=DIRECTION('ref_axis',(1.,0.,0.)) ;
#10399=DIRECTION('center_axis',(0.,0.,1.)) ;
#10400=DIRECTION('ref_axis',(1.,0.,0.)) ;
#10401=DIRECTION('center_axis',(0.,0.,1.)) ;
#10402=DIRECTION('ref_axis',(1.,0.,0.)) ;
#10403=DIRECTION('',(0.,0.,-1.)) ;
#10404=DIRECTION('center_axis',(0.,0.,-1.)) ;
#10405=DIRECTION('ref_axis',(-1.,0.,0.)) ;
#10406=DIRECTION('center_axis',(0.,0.,1.)) ;
#10407=DIRECTION('ref_axis',(1.,0.,0.)) ;
#13237=CARTESIAN_POINT('',(0.,0.,0.)) ;
#13238=CARTESIAN_POINT('Origin',(-1.,0.,-0.74)) ;
#13239=CARTESIAN_POINT('',(-1.26,-3.18408167778312E-17,-1.2)) ;
#13240=CARTESIAN_POINT('Origin',(-1.,0.,-1.2)) ;
#13241=CARTESIAN_POINT('',(-1.26,-3.18408167778312E-17,-0.18)) ;
#13242=CARTESIAN_POINT('',(-1.26,-3.18408167778312E-17,-0.74)) ;
#13243=CARTESIAN_POINT('Origin',(-1.,0.,-0.18)) ;
#13244=CARTESIAN_POINT('Origin',(-1.,0.,-0.18)) ;
#13245=CARTESIAN_POINT('Origin',(-1.,-0.7,0.4)) ;
#13246=CARTESIAN_POINT('',(-1.2,-0.7,0.5)) ;
#13247=CARTESIAN_POINT('',(-0.8,-0.7,0.5)) ;
#13248=CARTESIAN_POINT('',(-1.,-0.7,0.5)) ;
#13249=CARTESIAN_POINT('',(-1.2,-0.7,0.2)) ;
#13250=CARTESIAN_POINT('',(-1.2,-0.7,0.4)) ;
#13251=CARTESIAN_POINT('',(-0.8,-0.7,0.2)) ;
#13252=CARTESIAN_POINT('',(-1.,-0.7,0.2)) ;
#13253=CARTESIAN_POINT('',(-0.8,-0.7,0.4)) ;
#13254=CARTESIAN_POINT('Origin',(-0.8,-0.9,0.4)) ;
#13255=CARTESIAN_POINT('',(-0.8,-1.1,0.5)) ;
#13256=CARTESIAN_POINT('',(-0.8,-0.45,0.5)) ;
#13257=CARTESIAN_POINT('',(-0.8,-1.1,0.2)) ;
#13258=CARTESIAN_POINT('',(-0.8,-0.9,0.2)) ;
#13259=CARTESIAN_POINT('',(-0.8,-1.1,0.4)) ;
#13260=CARTESIAN_POINT('Origin',(-1.,-0.9,0.2)) ;
#13261=CARTESIAN_POINT('',(-1.2,-1.1,0.2)) ;
#13262=CARTESIAN_POINT('',(-1.2,-0.9,0.2)) ;
#13263=CARTESIAN_POINT('',(-1.,-1.1,0.2)) ;
#13264=CARTESIAN_POINT('Origin',(-1.,-1.1,0.4)) ;
#13265=CARTESIAN_POINT('',(-1.2,-1.1,0.5)) ;
#13266=CARTESIAN_POINT('',(-1.,-1.1,0.5)) ;
#13267=CARTESIAN_POINT('',(-1.2,-1.1,0.4)) ;
#13268=CARTESIAN_POINT('Origin',(-1.2,-0.9,0.4)) ;
#13269=CARTESIAN_POINT('',(-1.2,-0.45,0.5)) ;
#13270=CARTESIAN_POINT('Origin',(-1.77942286340599,0.65,0.4)) ;
#13271=CARTESIAN_POINT('',(-1.97942286340599,0.65,0.5)) ;
#13272=CARTESIAN_POINT('',(-1.579422863406,0.65,0.5)) ;
#13273=CARTESIAN_POINT('',(-1.389711431703,0.65,0.5)) ;
#13274=CARTESIAN_POINT('',(-1.97942286340599,0.65,0.2)) ;
#13275=CARTESIAN_POINT('',(-1.97942286340599,0.65,0.4)) ;
#13276=CARTESIAN_POINT('',(-1.579422863406,0.65,0.2)) ;
#13277=CARTESIAN_POINT('',(-1.77942286340599,0.65,0.2)) ;
#13278=CARTESIAN_POINT('',(-1.579422863406,0.65,0.4)) ;
#13279=CARTESIAN_POINT('Origin',(-1.579422863406,0.45,0.4)) ;
#13280=CARTESIAN_POINT('',(-1.579422863406,0.25,0.5)) ;
#13281=CARTESIAN_POINT('',(-1.57942286340599,0.225,0.5)) ;
#13282=CARTESIAN_POINT('',(-1.579422863406,0.25,0.2)) ;
#13283=CARTESIAN_POINT('',(-1.579422863406,0.45,0.2)) ;
#13284=CARTESIAN_POINT('',(-1.579422863406,0.25,0.4)) ;
#13285=CARTESIAN_POINT('Origin',(-1.77942286340599,0.45,0.2)) ;
#13286=CARTESIAN_POINT('',(-1.97942286340599,0.25,0.2)) ;
#13287=CARTESIAN_POINT('',(-1.97942286340599,0.45,0.2)) ;
#13288=CARTESIAN_POINT('',(-1.77942286340599,0.25,0.2)) ;
#13289=CARTESIAN_POINT('Origin',(-1.77942286340599,0.25,0.4)) ;
#13290=CARTESIAN_POINT('',(-1.97942286340599,0.25,0.5)) ;
#13291=CARTESIAN_POINT('',(-1.389711431703,0.25,0.5)) ;
#13292=CARTESIAN_POINT('',(-1.97942286340599,0.25,0.4)) ;
#13293=CARTESIAN_POINT('Origin',(-1.97942286340599,0.45,0.4)) ;
#13294=CARTESIAN_POINT('',(-1.979422863406,0.225,0.5)) ;
#13295=CARTESIAN_POINT('Origin',(-0.220577136594005,0.65,0.4)) ;
#13296=CARTESIAN_POINT('',(-0.420577136594005,0.65,0.5)) ;
#13297=CARTESIAN_POINT('',(-0.0205771365940052,0.65,0.5)) ;
#13298=CARTESIAN_POINT('',(-0.610288568297003,0.65,0.5)) ;
#13299=CARTESIAN_POINT('',(-0.420577136594005,0.65,0.2)) ;
#13300=CARTESIAN_POINT('',(-0.420577136594005,0.65,0.4)) ;
#13301=CARTESIAN_POINT('',(-0.0205771365940052,0.65,0.2)) ;
#13302=CARTESIAN_POINT('',(-0.220577136594005,0.65,0.2)) ;
#13303=CARTESIAN_POINT('',(-0.0205771365940052,0.65,0.4)) ;
#13304=CARTESIAN_POINT('Origin',(-0.0205771365940052,0.45,0.4)) ;
#13305=CARTESIAN_POINT('',(-0.0205771365940052,0.25,0.5)) ;
#13306=CARTESIAN_POINT('',(-0.0205771365940052,0.225,0.5)) ;
#13307=CARTESIAN_POINT('',(-0.0205771365940052,0.25,0.2)) ;
#13308=CARTESIAN_POINT('',(-0.0205771365940052,0.45,0.2)) ;
#13309=CARTESIAN_POINT('',(-0.0205771365940052,0.25,0.4)) ;
#13310=CARTESIAN_POINT('Origin',(-0.220577136594005,0.45,0.2)) ;
#13311=CARTESIAN_POINT('',(-0.420577136594005,0.25,0.2)) ;
#13312=CARTESIAN_POINT('',(-0.420577136594005,0.45,0.2)) ;
#13313=CARTESIAN_POINT('',(-0.220577136594005,0.25,0.2)) ;
#13314=CARTESIAN_POINT('Origin',(-0.220577136594005,0.25,0.4)) ;
#13315=CARTESIAN_POINT('',(-0.420577136594005,0.25,0.5)) ;
#13316=CARTESIAN_POINT('',(-0.610288568297003,0.25,0.5)) ;
#13317=CARTESIAN_POINT('',(-0.420577136594005,0.25,0.4)) ;
#13318=CARTESIAN_POINT('Origin',(-0.420577136594005,0.45,0.4)) ;
#13319=CARTESIAN_POINT('',(-0.420577136594005,0.225,0.5)) ;
#13320=CARTESIAN_POINT('Origin',(-1.,0.,-0.79)) ;
#13321=CARTESIAN_POINT('',(-1.69,8.45006291411674E-17,-0.28)) ;
#13322=CARTESIAN_POINT('Origin',(-1.,0.,-0.28)) ;
#13323=CARTESIAN_POINT('',(-1.69,8.45006291411674E-17,-1.2)) ;
#13324=CARTESIAN_POINT('',(-1.69,-8.45006291411674E-17,-0.79)) ;
#13325=CARTESIAN_POINT('Origin',(-1.,0.,-1.2)) ;
#13326=CARTESIAN_POINT('Origin',(-1.,0.,-0.79)) ;
#13327=CARTESIAN_POINT('',(-1.81,-9.91963907309356E-17,-1.2)) ;
#13328=CARTESIAN_POINT('Origin',(-1.,0.,-1.2)) ;
#13329=CARTESIAN_POINT('',(-1.81,-9.91963907309356E-17,-0.28)) ;
#13330=CARTESIAN_POINT('',(-1.81,-9.91963907309356E-17,-0.79)) ;
#13331=CARTESIAN_POINT('Origin',(-1.,0.,-0.28)) ;
#13332=CARTESIAN_POINT('Origin',(-1.,0.,-0.28)) ;
#13333=CARTESIAN_POINT('Origin',(-1.,0.,-1.2)) ;
#13334=CARTESIAN_POINT('',(-2.09,1.33486501107061E-16,-1.2)) ;
#13335=CARTESIAN_POINT('Origin',(-1.,0.,-1.2)) ;
#13336=CARTESIAN_POINT('Origin',(-1.,0.,-0.79)) ;
#13337=CARTESIAN_POINT('',(-2.09,1.33486501107061E-16,-0.28)) ;
#13338=CARTESIAN_POINT('Origin',(-1.,0.,-0.28)) ;
#13339=CARTESIAN_POINT('',(-2.09,-1.33486501107061E-16,-0.79)) ;
#13340=CARTESIAN_POINT('Origin',(-1.,0.,-0.79)) ;
#13341=CARTESIAN_POINT('',(-2.21,-1.4818226269683E-16,-1.2)) ;
#13342=CARTESIAN_POINT('Origin',(-1.,0.,-1.2)) ;
#13343=CARTESIAN_POINT('',(-2.21,-1.4818226269683E-16,-0.28)) ;
#13344=CARTESIAN_POINT('',(-2.21,-1.4818226269683E-16,-0.79)) ;
#13345=CARTESIAN_POINT('Origin',(-1.,0.,-0.28)) ;
#13346=CARTESIAN_POINT('Origin',(-1.,0.,-0.28)) ;
#13347=CARTESIAN_POINT('Origin',(-1.,0.,-1.2)) ;
#13348=CARTESIAN_POINT('',(-2.3,-1.59204083889156E-16,-1.2)) ;
#13349=CARTESIAN_POINT('Origin',(-1.,0.,-1.2)) ;
#13350=CARTESIAN_POINT('Origin',(-1.,0.,-0.35)) ;
#13351=CARTESIAN_POINT('',(-2.3,-1.59204083889156E-16,0.5)) ;
#13352=CARTESIAN_POINT('Origin',(-1.,0.,0.5)) ;
#13353=CARTESIAN_POINT('',(-2.3,-1.59204083889156E-16,-0.35)) ;
#13354=CARTESIAN_POINT('Origin',(-1.,0.,-1.2)) ;
#13355=CARTESIAN_POINT('Origin',(-1.,0.,0.5)) ;
#15404=UNCERTAINTY_MEASURE_WITH_UNIT(LENGTH_MEASURE(0.001),#15485,
'DISTANCE_ACCURACY_VALUE',
'Maximum model space distance between geometric entities at asserted c
onnectivities') ;
#15441=UNCERTAINTY_MEASURE_WITH_UNIT(LENGTH_MEASURE(0.001),#15485,
'DISTANCE_ACCURACY_VALUE',
'Maximum model space distance between geometric entities at asserted c
onnectivities') ;
#15447=(
GEOMETRIC_REPRESENTATION_CONTEXT(3)
GLOBAL_UNCERTAINTY_ASSIGNED_CONTEXT((#15404))
GLOBAL_UNIT_ASSIGNED_CONTEXT((#15485,#15487,#15488))
REPRESENTATION_CONTEXT('','3D')
) ;
#15484=(
GEOMETRIC_REPRESENTATION_CONTEXT(3)
GLOBAL_UNCERTAINTY_ASSIGNED_CONTEXT((#15441))
GLOBAL_UNIT_ASSIGNED_CONTEXT((#15485,#15487,#15488))
REPRESENTATION_CONTEXT('','3D')
) ;
#15485=(
LENGTH_UNIT()
NAMED_UNIT(*)
SI_UNIT(.CENTI.,.METRE.)
) ;
#15487=(
NAMED_UNIT(*)
PLANE_ANGLE_UNIT()
SI_UNIT($,.RADIAN.)
) ;
#15488=(
NAMED_UNIT(*)
SI_UNIT($,.STERADIAN.)
SOLID_ANGLE_UNIT()
) ;
#15494=SHAPE_DEFINITION_REPRESENTATION(#15538,#15623) ;
#15538=PRODUCT_DEFINITION_SHAPE('',$,#15666) ;
#15623=SHAPE_REPRESENTATION('',(#8799),#15447) ;
#15660=PRODUCT_DEFINITION_CONTEXT('part definition',#15788,'design') ;
#15666=PRODUCT_DEFINITION('STANDARD_3PIN_STRIX_CONNECTOR_BASE',
'STANDARD_3PIN_STRIX_CONNECTOR_BASE',#15708,#15660) ;
#15708=PRODUCT_DEFINITION_FORMATION('',$,#15795) ;
#15788=APPLICATION_CONTEXT(
'Core Data for Automotive Mechanical Design Process') ;
#15789=PRODUCT_CONTEXT('part definition',#15788,'mechanical') ;
#15795=PRODUCT('STANDARD_3PIN_STRIX_CONNECTOR_BASE',
'STANDARD_3PIN_STRIX_CONNECTOR_BASE',$,(#15789)) ;
#15833=PRESENTATION_STYLE_ASSIGNMENT((#15845)) ;
#15845=SURFACE_STYLE_USAGE(.BOTH.,#15857) ;
#15857=SURFACE_SIDE_STYLE('',(#15869)) ;
#15869=SURFACE_STYLE_FILL_AREA(#15881) ;
#15881=FILL_AREA_STYLE('Nylon 6-6 (White)',(#15893)) ;
#15893=FILL_AREA_STYLE_COLOUR('Nylon 6-6 (White)',#15905) ;
#15905=COLOUR_RGB('Nylon 6-6 (White)', 0.31764706, 0.68627451, 0.89019608) ;
ENDSEC;
END-ISO-10303-21;
